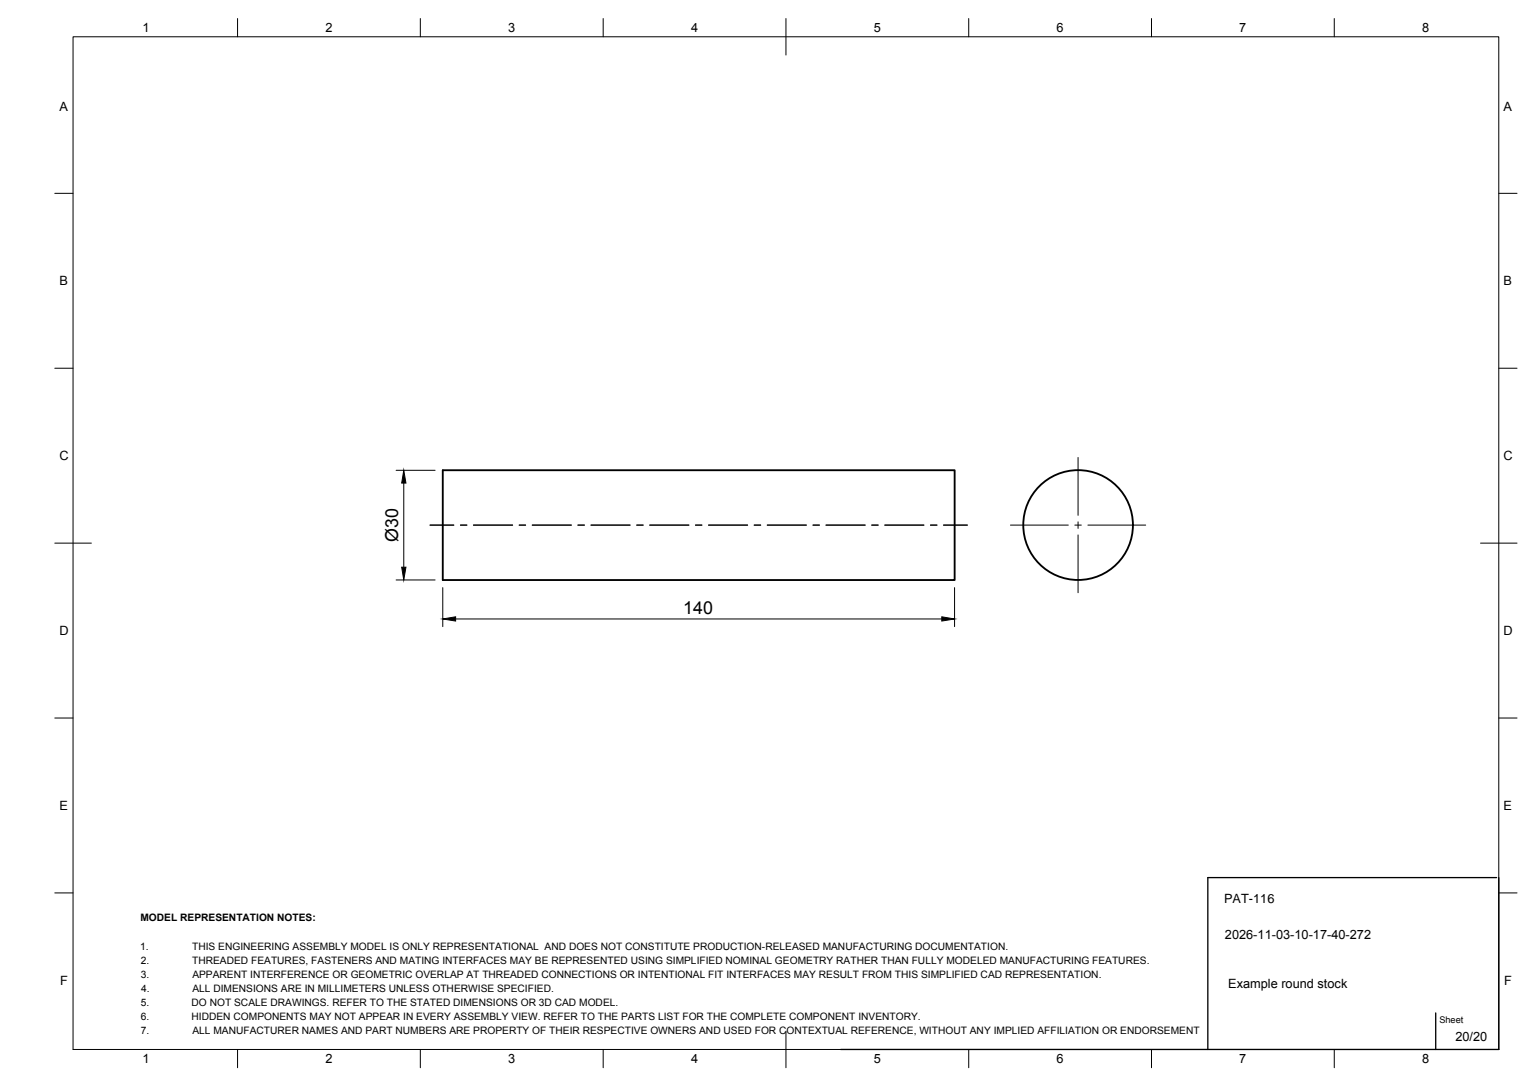
ISO-10303-21;
HEADER;
/* Generated by software containing ST-Developer
 * from STEP Tools, Inc. (www.steptools.com) 
 */

FILE_DESCRIPTION(
/* description */ ('V-block with clamp strap'),
/* implementation_level */ '2;1');

FILE_NAME(
/* name */ 'Example round stock.step',
/* time_stamp */ '2026-10-27T10:50:53-07:00',
/* author */ (''),
/* organization */ (''),
/* preprocessor_version */ 'ST-DEVELOPER v20.2',
/* originating_system */ 'Autodesk Translation Framework v15.17.0.0',
/* authorisation */ '');

FILE_SCHEMA (('AUTOMOTIVE_DESIGN { 1 0 10303 214 3 1 1 }'));
ENDSEC;

DATA;
#10=MECHANICAL_DESIGN_GEOMETRIC_PRESENTATION_REPRESENTATION('',(#286),#7344);
#244=SHAPE_REPRESENTATION_RELATIONSHIP('SRR','None',#7464,#265);
#265=ADVANCED_BREP_SHAPE_REPRESENTATION('',(#304),#7343);
#286=STYLED_ITEM('',(#7624),#304);
#304=MANIFOLD_SOLID_BREP('Body1',#4171);
#503=CIRCLE('',#4835,1.5);
#504=CIRCLE('',#4836,1.5);
#561=CYLINDRICAL_SURFACE('',#4834,1.5);
#799=FACE_OUTER_BOUND('',#1110,.T.);
#800=FACE_OUTER_BOUND('',#1111,.T.);
#801=FACE_OUTER_BOUND('',#1112,.T.);
#1110=EDGE_LOOP('',(#3734,#3735,#3736,#3737));
#1111=EDGE_LOOP('',(#3738));
#1112=EDGE_LOOP('',(#3739));
#1477=LINE('',#7285,#1842);
#1842=VECTOR('',#6071,1.5);
#2172=VERTEX_POINT('',#7282);
#2173=VERTEX_POINT('',#7284);
#2693=EDGE_CURVE('',#2172,#2172,#503,.T.);
#2694=EDGE_CURVE('',#2172,#2173,#1477,.T.);
#2695=EDGE_CURVE('',#2173,#2173,#504,.T.);
#3734=ORIENTED_EDGE('',*,*,#2693,.F.);
#3735=ORIENTED_EDGE('',*,*,#2694,.T.);
#3736=ORIENTED_EDGE('',*,*,#2695,.T.);
#3737=ORIENTED_EDGE('',*,*,#2694,.F.);
#3738=ORIENTED_EDGE('',*,*,#2693,.T.);
#3739=ORIENTED_EDGE('',*,*,#2695,.F.);
#3906=PLANE('',#4837);
#3907=PLANE('',#4838);
#4145=ADVANCED_FACE('',(#799),#561,.T.);
#4146=ADVANCED_FACE('',(#800),#3906,.T.);
#4147=ADVANCED_FACE('',(#801),#3907,.F.);
#4171=CLOSED_SHELL('',(#4145,#4146,#4147));
#4833=AXIS2_PLACEMENT_3D('',#7280,#6065,#6066);
#4834=AXIS2_PLACEMENT_3D('',#7281,#6067,#6068);
#4835=AXIS2_PLACEMENT_3D('',#7283,#6069,#6070);
#4836=AXIS2_PLACEMENT_3D('',#7286,#6072,#6073);
#4837=AXIS2_PLACEMENT_3D('',#7287,#6074,#6075);
#4838=AXIS2_PLACEMENT_3D('',#7288,#6076,#6077);
#6065=DIRECTION('axis',(0.,0.,1.));
#6066=DIRECTION('refdir',(1.,0.,0.));
#6067=DIRECTION('center_axis',(1.,0.,0.));
#6068=DIRECTION('ref_axis',(0.,0.,-1.));
#6069=DIRECTION('center_axis',(1.,0.,0.));
#6070=DIRECTION('ref_axis',(0.,0.,-1.));
#6071=DIRECTION('',(-1.,0.,0.));
#6072=DIRECTION('center_axis',(1.,0.,0.));
#6073=DIRECTION('ref_axis',(0.,0.,-1.));
#6074=DIRECTION('center_axis',(1.,0.,0.));
#6075=DIRECTION('ref_axis',(0.,0.,-1.));
#6076=DIRECTION('center_axis',(1.,0.,0.));
#6077=DIRECTION('ref_axis',(0.,0.,-1.));
#7280=CARTESIAN_POINT('',(0.,0.,0.));
#7281=CARTESIAN_POINT('Origin',(3.,0.,4.62132034355964));
#7282=CARTESIAN_POINT('',(17.,-1.83697019872103E-16,6.12132034355964));
#7283=CARTESIAN_POINT('Origin',(17.,0.,4.62132034355964));
#7284=CARTESIAN_POINT('',(3.,-1.83697019872103E-16,6.12132034355964));
#7285=CARTESIAN_POINT('',(3.,-1.83697019872103E-16,6.12132034355964));
#7286=CARTESIAN_POINT('Origin',(3.,0.,4.62132034355964));
#7287=CARTESIAN_POINT('Origin',(17.,0.,4.62132034355964));
#7288=CARTESIAN_POINT('Origin',(3.,0.,4.62132034355964));
#7317=UNCERTAINTY_MEASURE_WITH_UNIT(LENGTH_MEASURE(0.001),#7345,
'DISTANCE_ACCURACY_VALUE',
'Maximum model space distance between geometric entities at asserted c
onnectivities');
#7318=UNCERTAINTY_MEASURE_WITH_UNIT(LENGTH_MEASURE(0.001),#7345,
'DISTANCE_ACCURACY_VALUE',
'Maximum model space distance between geometric entities at asserted c
onnectivities');
#7343=(
GEOMETRIC_REPRESENTATION_CONTEXT(3)
GLOBAL_UNCERTAINTY_ASSIGNED_CONTEXT((#7317))
GLOBAL_UNIT_ASSIGNED_CONTEXT((#7345,#7347,#7348))
REPRESENTATION_CONTEXT('','3D')
);
#7344=(
GEOMETRIC_REPRESENTATION_CONTEXT(3)
GLOBAL_UNCERTAINTY_ASSIGNED_CONTEXT((#7318))
GLOBAL_UNIT_ASSIGNED_CONTEXT((#7345,#7347,#7348))
REPRESENTATION_CONTEXT('','3D')
);
#7345=(
LENGTH_UNIT()
NAMED_UNIT(*)
SI_UNIT(.CENTI.,.METRE.)
);
#7347=(
NAMED_UNIT(*)
PLANE_ANGLE_UNIT()
SI_UNIT($,.RADIAN.)
);
#7348=(
NAMED_UNIT(*)
SI_UNIT($,.STERADIAN.)
SOLID_ANGLE_UNIT()
);
#7373=SHAPE_DEFINITION_REPRESENTATION(#7435,#7464);
#7435=PRODUCT_DEFINITION_SHAPE('',$,#7490);
#7464=SHAPE_REPRESENTATION('',(#4833),#7343);
#7465=PRODUCT_DEFINITION_CONTEXT('part definition',#7542,'design');
#7490=PRODUCT_DEFINITION('Example round stock','Example round stock',
#7515,#7465);
#7515=PRODUCT_DEFINITION_FORMATION('',$,#7568);
#7542=APPLICATION_CONTEXT(
'Core Data for Automotive Mechanical Design Process');
#7543=PRODUCT_CONTEXT('part definition',#7542,'mechanical');
#7568=PRODUCT('Example round stock','Example round stock',
'Example round stock',(#7543));
#7618=COLOUR_RGB('Sky Blue',0.24,0.69,0.87);
#7619=FILL_AREA_STYLE_COLOUR('',#7618);
#7620=FILL_AREA_STYLE('',(#7619));
#7621=SURFACE_STYLE_FILL_AREA(#7620);
#7622=SURFACE_SIDE_STYLE('',(#7621));
#7623=SURFACE_STYLE_USAGE(.BOTH.,#7622);
#7624=PRESENTATION_STYLE_ASSIGNMENT((#7623));
ENDSEC;
END-ISO-10303-21;
